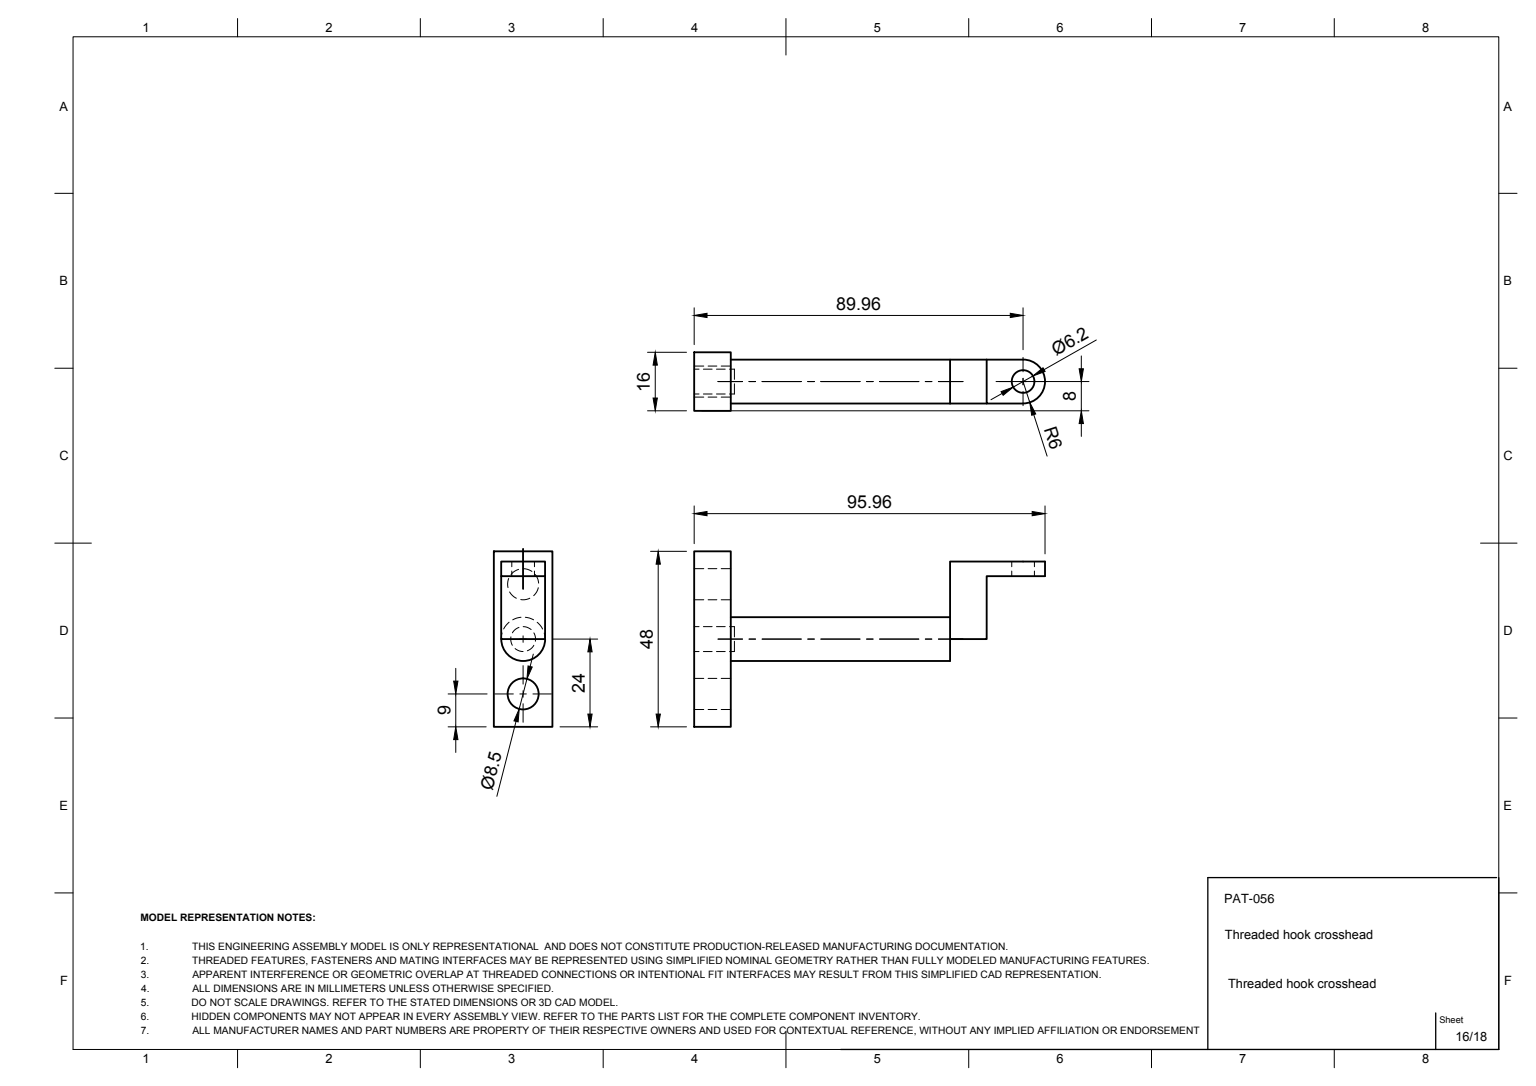
ISO-10303-21;
HEADER;
/* Generated by software containing ST-Developer
 * from STEP Tools, Inc. (www.steptools.com) 
 */

FILE_DESCRIPTION(
/* description */ ('Hook toggle clamp'),
/* implementation_level */ '2;1');

FILE_NAME(
/* name */ 'Threaded hook crosshead.step',
/* time_stamp */ '2026-10-27T21:56:56-07:00',
/* author */ (''),
/* organization */ (''),
/* preprocessor_version */ 'ST-DEVELOPER v20.2',
/* originating_system */ 'Autodesk Translation Framework v15.17.0.0',
/* authorisation */ '');

FILE_SCHEMA (('AUTOMOTIVE_DESIGN { 1 0 10303 214 3 1 1 }'));
ENDSEC;

DATA;
#10=MECHANICAL_DESIGN_GEOMETRIC_PRESENTATION_REPRESENTATION('',(#198),#5458);
#164=SHAPE_REPRESENTATION_RELATIONSHIP('SRR','None',#5548,#181);
#181=ADVANCED_BREP_SHAPE_REPRESENTATION('',(#214),#5450);
#198=STYLED_ITEM('',(#5731),#214);
#214=MANIFOLD_SOLID_BREP('Body1',#2980);
#259=FACE_BOUND('',#719,.T.);
#260=FACE_BOUND('',#720,.T.);
#261=FACE_BOUND('',#721,.T.);
#262=FACE_BOUND('',#727,.T.);
#263=FACE_BOUND('',#728,.T.);
#264=FACE_BOUND('',#729,.T.);
#265=FACE_BOUND('',#733,.T.);
#266=FACE_BOUND('',#740,.T.);
#356=PLANE('',#3372);
#357=PLANE('',#3379);
#358=PLANE('',#3381);
#359=PLANE('',#3382);
#360=PLANE('',#3383);
#361=PLANE('',#3384);
#362=PLANE('',#3385);
#363=PLANE('',#3392);
#364=PLANE('',#3393);
#365=PLANE('',#3394);
#366=PLANE('',#3395);
#367=PLANE('',#3396);
#368=PLANE('',#3397);
#369=PLANE('',#3399);
#370=PLANE('',#3400);
#504=FACE_OUTER_BOUND('',#714,.T.);
#505=FACE_OUTER_BOUND('',#715,.T.);
#506=FACE_OUTER_BOUND('',#716,.T.);
#507=FACE_OUTER_BOUND('',#717,.T.);
#508=FACE_OUTER_BOUND('',#718,.T.);
#509=FACE_OUTER_BOUND('',#722,.T.);
#510=FACE_OUTER_BOUND('',#723,.T.);
#511=FACE_OUTER_BOUND('',#724,.T.);
#512=FACE_OUTER_BOUND('',#725,.T.);
#513=FACE_OUTER_BOUND('',#726,.T.);
#514=FACE_OUTER_BOUND('',#730,.T.);
#515=FACE_OUTER_BOUND('',#731,.T.);
#516=FACE_OUTER_BOUND('',#732,.T.);
#517=FACE_OUTER_BOUND('',#734,.T.);
#518=FACE_OUTER_BOUND('',#735,.T.);
#519=FACE_OUTER_BOUND('',#736,.T.);
#520=FACE_OUTER_BOUND('',#737,.T.);
#521=FACE_OUTER_BOUND('',#738,.T.);
#522=FACE_OUTER_BOUND('',#739,.T.);
#523=FACE_OUTER_BOUND('',#741,.T.);
#524=FACE_OUTER_BOUND('',#742,.T.);
#714=EDGE_LOOP('',(#2497,#2498,#2499,#2500));
#715=EDGE_LOOP('',(#2501));
#716=EDGE_LOOP('',(#2502,#2503,#2504,#2505));
#717=EDGE_LOOP('',(#2506,#2507,#2508,#2509));
#718=EDGE_LOOP('',(#2510,#2511,#2512,#2513));
#719=EDGE_LOOP('',(#2514));
#720=EDGE_LOOP('',(#2515));
#721=EDGE_LOOP('',(#2516));
#722=EDGE_LOOP('',(#2517,#2518,#2519,#2520));
#723=EDGE_LOOP('',(#2521,#2522,#2523,#2524));
#724=EDGE_LOOP('',(#2525,#2526,#2527,#2528));
#725=EDGE_LOOP('',(#2529,#2530,#2531,#2532));
#726=EDGE_LOOP('',(#2533,#2534,#2535,#2536));
#727=EDGE_LOOP('',(#2537));
#728=EDGE_LOOP('',(#2538));
#729=EDGE_LOOP('',(#2539));
#730=EDGE_LOOP('',(#2540,#2541,#2542,#2543));
#731=EDGE_LOOP('',(#2544,#2545,#2546,#2547));
#732=EDGE_LOOP('',(#2548,#2549,#2550,#2551));
#733=EDGE_LOOP('',(#2552));
#734=EDGE_LOOP('',(#2553,#2554,#2555,#2556));
#735=EDGE_LOOP('',(#2557,#2558,#2559,#2560));
#736=EDGE_LOOP('',(#2561,#2562,#2563,#2564,#2565,#2566));
#737=EDGE_LOOP('',(#2567,#2568,#2569,#2570,#2571,#2572));
#738=EDGE_LOOP('',(#2573,#2574,#2575,#2576));
#739=EDGE_LOOP('',(#2577,#2578,#2579,#2580));
#740=EDGE_LOOP('',(#2581));
#741=EDGE_LOOP('',(#2582,#2583));
#742=EDGE_LOOP('',(#2584,#2585,#2586,#2587,#2588));
#971=LINE('',#4973,#1208);
#972=LINE('',#4980,#1209);
#973=LINE('',#4986,#1210);
#974=LINE('',#4991,#1211);
#975=LINE('',#4993,#1212);
#976=LINE('',#4995,#1213);
#977=LINE('',#4996,#1214);
#978=LINE('',#5001,#1215);
#979=LINE('',#5003,#1216);
#980=LINE('',#5004,#1217);
#981=LINE('',#5007,#1218);
#982=LINE('',#5008,#1219);
#983=LINE('',#5011,#1220);
#984=LINE('',#5012,#1221);
#985=LINE('',#5014,#1222);
#986=LINE('',#5020,#1223);
#987=LINE('',#5025,#1224);
#988=LINE('',#5029,#1225);
#989=LINE('',#5033,#1226);
#990=LINE('',#5035,#1227);
#991=LINE('',#5036,#1228);
#992=LINE('',#5039,#1229);
#993=LINE('',#5041,#1230);
#994=LINE('',#5042,#1231);
#995=LINE('',#5045,#1232);
#996=LINE('',#5047,#1233);
#997=LINE('',#5048,#1234);
#998=LINE('',#5051,#1235);
#999=LINE('',#5052,#1236);
#1000=LINE('',#5055,#1237);
#1001=LINE('',#5056,#1238);
#1002=LINE('',#5058,#1239);
#1003=LINE('',#5064,#1240);
#1208=VECTOR('',#4077,0.34);
#1209=VECTOR('',#4086,0.425);
#1210=VECTOR('',#4093,0.425);
#1211=VECTOR('',#4098,1.);
#1212=VECTOR('',#4099,1.);
#1213=VECTOR('',#4100,1.);
#1214=VECTOR('',#4101,1.);
#1215=VECTOR('',#4106,1.);
#1216=VECTOR('',#4107,1.);
#1217=VECTOR('',#4108,1.);
#1218=VECTOR('',#4111,1.);
#1219=VECTOR('',#4112,1.);
#1220=VECTOR('',#4115,1.);
#1221=VECTOR('',#4116,1.);
#1222=VECTOR('',#4119,1.);
#1223=VECTOR('',#4126,0.31);
#1224=VECTOR('',#4131,1.);
#1225=VECTOR('',#4134,1.);
#1226=VECTOR('',#4139,1.);
#1227=VECTOR('',#4140,1.);
#1228=VECTOR('',#4141,1.);
#1229=VECTOR('',#4144,1.);
#1230=VECTOR('',#4145,1.);
#1231=VECTOR('',#4146,1.);
#1232=VECTOR('',#4149,1.);
#1233=VECTOR('',#4150,1.);
#1234=VECTOR('',#4151,1.);
#1235=VECTOR('',#4154,1.);
#1236=VECTOR('',#4155,1.);
#1237=VECTOR('',#4158,1.);
#1238=VECTOR('',#4159,1.);
#1239=VECTOR('',#4162,1.);
#1240=VECTOR('',#4173,0.6);
#1335=CIRCLE('',#3370,0.34);
#1336=CIRCLE('',#3371,0.34);
#1337=CIRCLE('',#3374,0.425);
#1338=CIRCLE('',#3375,0.425);
#1339=CIRCLE('',#3377,0.425);
#1340=CIRCLE('',#3378,0.425);
#1341=CIRCLE('',#3380,0.6);
#1342=CIRCLE('',#3387,0.31);
#1343=CIRCLE('',#3388,0.31);
#1344=CIRCLE('',#3390,0.6);
#1345=CIRCLE('',#3391,0.6);
#1346=CIRCLE('',#3398,0.6);
#1347=CIRCLE('',#3401,0.6);
#1546=VERTEX_POINT('',#4970);
#1547=VERTEX_POINT('',#4972);
#1548=VERTEX_POINT('',#4977);
#1549=VERTEX_POINT('',#4979);
#1550=VERTEX_POINT('',#4983);
#1551=VERTEX_POINT('',#4985);
#1552=VERTEX_POINT('',#4989);
#1553=VERTEX_POINT('',#4990);
#1554=VERTEX_POINT('',#4992);
#1555=VERTEX_POINT('',#4994);
#1556=VERTEX_POINT('',#4997);
#1557=VERTEX_POINT('',#5000);
#1558=VERTEX_POINT('',#5002);
#1559=VERTEX_POINT('',#5006);
#1560=VERTEX_POINT('',#5010);
#1561=VERTEX_POINT('',#5017);
#1562=VERTEX_POINT('',#5019);
#1563=VERTEX_POINT('',#5023);
#1564=VERTEX_POINT('',#5024);
#1565=VERTEX_POINT('',#5026);
#1566=VERTEX_POINT('',#5028);
#1567=VERTEX_POINT('',#5032);
#1568=VERTEX_POINT('',#5034);
#1569=VERTEX_POINT('',#5038);
#1570=VERTEX_POINT('',#5040);
#1571=VERTEX_POINT('',#5044);
#1572=VERTEX_POINT('',#5046);
#1573=VERTEX_POINT('',#5050);
#1574=VERTEX_POINT('',#5054);
#1875=EDGE_CURVE('',#1546,#1546,#1335,.T.);
#1876=EDGE_CURVE('',#1546,#1547,#971,.T.);
#1877=EDGE_CURVE('',#1547,#1547,#1336,.T.);
#1878=EDGE_CURVE('',#1548,#1548,#1337,.T.);
#1879=EDGE_CURVE('',#1548,#1549,#972,.T.);
#1880=EDGE_CURVE('',#1549,#1549,#1338,.T.);
#1881=EDGE_CURVE('',#1550,#1550,#1339,.T.);
#1882=EDGE_CURVE('',#1550,#1551,#973,.T.);
#1883=EDGE_CURVE('',#1551,#1551,#1340,.T.);
#1884=EDGE_CURVE('',#1552,#1553,#974,.T.);
#1885=EDGE_CURVE('',#1554,#1552,#975,.T.);
#1886=EDGE_CURVE('',#1555,#1554,#976,.T.);
#1887=EDGE_CURVE('',#1553,#1555,#977,.T.);
#1888=EDGE_CURVE('',#1556,#1556,#1341,.T.);
#1889=EDGE_CURVE('',#1552,#1557,#978,.T.);
#1890=EDGE_CURVE('',#1558,#1557,#979,.T.);
#1891=EDGE_CURVE('',#1554,#1558,#980,.T.);
#1892=EDGE_CURVE('',#1559,#1558,#981,.T.);
#1893=EDGE_CURVE('',#1555,#1559,#982,.T.);
#1894=EDGE_CURVE('',#1560,#1559,#983,.T.);
#1895=EDGE_CURVE('',#1553,#1560,#984,.T.);
#1896=EDGE_CURVE('',#1557,#1560,#985,.T.);
#1897=EDGE_CURVE('',#1561,#1561,#1342,.T.);
#1898=EDGE_CURVE('',#1561,#1562,#986,.T.);
#1899=EDGE_CURVE('',#1562,#1562,#1343,.T.);
#1900=EDGE_CURVE('',#1563,#1564,#987,.T.);
#1901=EDGE_CURVE('',#1565,#1564,#1344,.T.);
#1902=EDGE_CURVE('',#1566,#1565,#988,.T.);
#1903=EDGE_CURVE('',#1566,#1563,#1345,.T.);
#1904=EDGE_CURVE('',#1566,#1567,#989,.T.);
#1905=EDGE_CURVE('',#1567,#1568,#990,.T.);
#1906=EDGE_CURVE('',#1568,#1563,#991,.T.);
#1907=EDGE_CURVE('',#1569,#1567,#992,.T.);
#1908=EDGE_CURVE('',#1570,#1569,#993,.T.);
#1909=EDGE_CURVE('',#1570,#1568,#994,.T.);
#1910=EDGE_CURVE('',#1571,#1570,#995,.T.);
#1911=EDGE_CURVE('',#1569,#1572,#996,.T.);
#1912=EDGE_CURVE('',#1571,#1572,#997,.T.);
#1913=EDGE_CURVE('',#1573,#1565,#998,.T.);
#1914=EDGE_CURVE('',#1572,#1573,#999,.T.);
#1915=EDGE_CURVE('',#1564,#1574,#1000,.T.);
#1916=EDGE_CURVE('',#1571,#1574,#1001,.T.);
#1917=EDGE_CURVE('',#1574,#1573,#1002,.T.);
#1918=EDGE_CURVE('',#1572,#1571,#1346,.T.);
#1919=EDGE_CURVE('',#1571,#1572,#1347,.T.);
#1920=EDGE_CURVE('',#1556,#1571,#1003,.T.);
#2497=ORIENTED_EDGE('',*,*,#1875,.F.);
#2498=ORIENTED_EDGE('',*,*,#1876,.T.);
#2499=ORIENTED_EDGE('',*,*,#1877,.F.);
#2500=ORIENTED_EDGE('',*,*,#1876,.F.);
#2501=ORIENTED_EDGE('',*,*,#1875,.T.);
#2502=ORIENTED_EDGE('',*,*,#1878,.F.);
#2503=ORIENTED_EDGE('',*,*,#1879,.T.);
#2504=ORIENTED_EDGE('',*,*,#1880,.F.);
#2505=ORIENTED_EDGE('',*,*,#1879,.F.);
#2506=ORIENTED_EDGE('',*,*,#1881,.F.);
#2507=ORIENTED_EDGE('',*,*,#1882,.T.);
#2508=ORIENTED_EDGE('',*,*,#1883,.F.);
#2509=ORIENTED_EDGE('',*,*,#1882,.F.);
#2510=ORIENTED_EDGE('',*,*,#1884,.F.);
#2511=ORIENTED_EDGE('',*,*,#1885,.F.);
#2512=ORIENTED_EDGE('',*,*,#1886,.F.);
#2513=ORIENTED_EDGE('',*,*,#1887,.F.);
#2514=ORIENTED_EDGE('',*,*,#1878,.T.);
#2515=ORIENTED_EDGE('',*,*,#1881,.T.);
#2516=ORIENTED_EDGE('',*,*,#1888,.T.);
#2517=ORIENTED_EDGE('',*,*,#1885,.T.);
#2518=ORIENTED_EDGE('',*,*,#1889,.T.);
#2519=ORIENTED_EDGE('',*,*,#1890,.F.);
#2520=ORIENTED_EDGE('',*,*,#1891,.F.);
#2521=ORIENTED_EDGE('',*,*,#1886,.T.);
#2522=ORIENTED_EDGE('',*,*,#1891,.T.);
#2523=ORIENTED_EDGE('',*,*,#1892,.F.);
#2524=ORIENTED_EDGE('',*,*,#1893,.F.);
#2525=ORIENTED_EDGE('',*,*,#1887,.T.);
#2526=ORIENTED_EDGE('',*,*,#1893,.T.);
#2527=ORIENTED_EDGE('',*,*,#1894,.F.);
#2528=ORIENTED_EDGE('',*,*,#1895,.F.);
#2529=ORIENTED_EDGE('',*,*,#1884,.T.);
#2530=ORIENTED_EDGE('',*,*,#1895,.T.);
#2531=ORIENTED_EDGE('',*,*,#1896,.F.);
#2532=ORIENTED_EDGE('',*,*,#1889,.F.);
#2533=ORIENTED_EDGE('',*,*,#1896,.T.);
#2534=ORIENTED_EDGE('',*,*,#1894,.T.);
#2535=ORIENTED_EDGE('',*,*,#1892,.T.);
#2536=ORIENTED_EDGE('',*,*,#1890,.T.);
#2537=ORIENTED_EDGE('',*,*,#1877,.T.);
#2538=ORIENTED_EDGE('',*,*,#1880,.T.);
#2539=ORIENTED_EDGE('',*,*,#1883,.T.);
#2540=ORIENTED_EDGE('',*,*,#1897,.F.);
#2541=ORIENTED_EDGE('',*,*,#1898,.T.);
#2542=ORIENTED_EDGE('',*,*,#1899,.F.);
#2543=ORIENTED_EDGE('',*,*,#1898,.F.);
#2544=ORIENTED_EDGE('',*,*,#1900,.T.);
#2545=ORIENTED_EDGE('',*,*,#1901,.F.);
#2546=ORIENTED_EDGE('',*,*,#1902,.F.);
#2547=ORIENTED_EDGE('',*,*,#1903,.T.);
#2548=ORIENTED_EDGE('',*,*,#1904,.T.);
#2549=ORIENTED_EDGE('',*,*,#1905,.T.);
#2550=ORIENTED_EDGE('',*,*,#1906,.T.);
#2551=ORIENTED_EDGE('',*,*,#1903,.F.);
#2552=ORIENTED_EDGE('',*,*,#1897,.T.);
#2553=ORIENTED_EDGE('',*,*,#1905,.F.);
#2554=ORIENTED_EDGE('',*,*,#1907,.F.);
#2555=ORIENTED_EDGE('',*,*,#1908,.F.);
#2556=ORIENTED_EDGE('',*,*,#1909,.T.);
#2557=ORIENTED_EDGE('',*,*,#1910,.T.);
#2558=ORIENTED_EDGE('',*,*,#1908,.T.);
#2559=ORIENTED_EDGE('',*,*,#1911,.T.);
#2560=ORIENTED_EDGE('',*,*,#1912,.F.);
#2561=ORIENTED_EDGE('',*,*,#1904,.F.);
#2562=ORIENTED_EDGE('',*,*,#1902,.T.);
#2563=ORIENTED_EDGE('',*,*,#1913,.F.);
#2564=ORIENTED_EDGE('',*,*,#1914,.F.);
#2565=ORIENTED_EDGE('',*,*,#1911,.F.);
#2566=ORIENTED_EDGE('',*,*,#1907,.T.);
#2567=ORIENTED_EDGE('',*,*,#1915,.F.);
#2568=ORIENTED_EDGE('',*,*,#1900,.F.);
#2569=ORIENTED_EDGE('',*,*,#1906,.F.);
#2570=ORIENTED_EDGE('',*,*,#1909,.F.);
#2571=ORIENTED_EDGE('',*,*,#1910,.F.);
#2572=ORIENTED_EDGE('',*,*,#1916,.T.);
#2573=ORIENTED_EDGE('',*,*,#1914,.T.);
#2574=ORIENTED_EDGE('',*,*,#1917,.F.);
#2575=ORIENTED_EDGE('',*,*,#1916,.F.);
#2576=ORIENTED_EDGE('',*,*,#1918,.F.);
#2577=ORIENTED_EDGE('',*,*,#1915,.T.);
#2578=ORIENTED_EDGE('',*,*,#1917,.T.);
#2579=ORIENTED_EDGE('',*,*,#1913,.T.);
#2580=ORIENTED_EDGE('',*,*,#1901,.T.);
#2581=ORIENTED_EDGE('',*,*,#1899,.T.);
#2582=ORIENTED_EDGE('',*,*,#1912,.T.);
#2583=ORIENTED_EDGE('',*,*,#1919,.F.);
#2584=ORIENTED_EDGE('',*,*,#1888,.F.);
#2585=ORIENTED_EDGE('',*,*,#1920,.T.);
#2586=ORIENTED_EDGE('',*,*,#1919,.T.);
#2587=ORIENTED_EDGE('',*,*,#1918,.T.);
#2588=ORIENTED_EDGE('',*,*,#1920,.F.);
#2778=CYLINDRICAL_SURFACE('',#3369,0.34);
#2779=CYLINDRICAL_SURFACE('',#3373,0.425);
#2780=CYLINDRICAL_SURFACE('',#3376,0.425);
#2781=CYLINDRICAL_SURFACE('',#3386,0.31);
#2782=CYLINDRICAL_SURFACE('',#3389,0.6);
#2783=CYLINDRICAL_SURFACE('',#3402,0.6);
#2908=ADVANCED_FACE('',(#504),#2778,.F.);
#2909=ADVANCED_FACE('',(#505),#356,.T.);
#2910=ADVANCED_FACE('',(#506),#2779,.F.);
#2911=ADVANCED_FACE('',(#507),#2780,.F.);
#2912=ADVANCED_FACE('',(#508,#259,#260,#261),#357,.F.);
#2913=ADVANCED_FACE('',(#509),#358,.T.);
#2914=ADVANCED_FACE('',(#510),#359,.T.);
#2915=ADVANCED_FACE('',(#511),#360,.T.);
#2916=ADVANCED_FACE('',(#512),#361,.T.);
#2917=ADVANCED_FACE('',(#513,#262,#263,#264),#362,.T.);
#2918=ADVANCED_FACE('',(#514),#2781,.F.);
#2919=ADVANCED_FACE('',(#515),#2782,.T.);
#2920=ADVANCED_FACE('',(#516,#265),#363,.F.);
#2921=ADVANCED_FACE('',(#517),#364,.T.);
#2922=ADVANCED_FACE('',(#518),#365,.F.);
#2923=ADVANCED_FACE('',(#519),#366,.T.);
#2924=ADVANCED_FACE('',(#520),#367,.T.);
#2925=ADVANCED_FACE('',(#521),#368,.T.);
#2926=ADVANCED_FACE('',(#522,#266),#369,.T.);
#2927=ADVANCED_FACE('',(#523),#370,.F.);
#2928=ADVANCED_FACE('',(#524),#2783,.T.);
#2980=CLOSED_SHELL('',(#2908,#2909,#2910,#2911,#2912,#2913,#2914,#2915,
#2916,#2917,#2918,#2919,#2920,#2921,#2922,#2923,#2924,#2925,#2926,#2927,
#2928));
#3368=AXIS2_PLACEMENT_3D('',#4968,#4071,#4072);
#3369=AXIS2_PLACEMENT_3D('',#4969,#4073,#4074);
#3370=AXIS2_PLACEMENT_3D('',#4971,#4075,#4076);
#3371=AXIS2_PLACEMENT_3D('',#4974,#4078,#4079);
#3372=AXIS2_PLACEMENT_3D('',#4975,#4080,#4081);
#3373=AXIS2_PLACEMENT_3D('',#4976,#4082,#4083);
#3374=AXIS2_PLACEMENT_3D('',#4978,#4084,#4085);
#3375=AXIS2_PLACEMENT_3D('',#4981,#4087,#4088);
#3376=AXIS2_PLACEMENT_3D('',#4982,#4089,#4090);
#3377=AXIS2_PLACEMENT_3D('',#4984,#4091,#4092);
#3378=AXIS2_PLACEMENT_3D('',#4987,#4094,#4095);
#3379=AXIS2_PLACEMENT_3D('',#4988,#4096,#4097);
#3380=AXIS2_PLACEMENT_3D('',#4998,#4102,#4103);
#3381=AXIS2_PLACEMENT_3D('',#4999,#4104,#4105);
#3382=AXIS2_PLACEMENT_3D('',#5005,#4109,#4110);
#3383=AXIS2_PLACEMENT_3D('',#5009,#4113,#4114);
#3384=AXIS2_PLACEMENT_3D('',#5013,#4117,#4118);
#3385=AXIS2_PLACEMENT_3D('',#5015,#4120,#4121);
#3386=AXIS2_PLACEMENT_3D('',#5016,#4122,#4123);
#3387=AXIS2_PLACEMENT_3D('',#5018,#4124,#4125);
#3388=AXIS2_PLACEMENT_3D('',#5021,#4127,#4128);
#3389=AXIS2_PLACEMENT_3D('',#5022,#4129,#4130);
#3390=AXIS2_PLACEMENT_3D('',#5027,#4132,#4133);
#3391=AXIS2_PLACEMENT_3D('',#5030,#4135,#4136);
#3392=AXIS2_PLACEMENT_3D('',#5031,#4137,#4138);
#3393=AXIS2_PLACEMENT_3D('',#5037,#4142,#4143);
#3394=AXIS2_PLACEMENT_3D('',#5043,#4147,#4148);
#3395=AXIS2_PLACEMENT_3D('',#5049,#4152,#4153);
#3396=AXIS2_PLACEMENT_3D('',#5053,#4156,#4157);
#3397=AXIS2_PLACEMENT_3D('',#5057,#4160,#4161);
#3398=AXIS2_PLACEMENT_3D('',#5059,#4163,#4164);
#3399=AXIS2_PLACEMENT_3D('',#5060,#4165,#4166);
#3400=AXIS2_PLACEMENT_3D('',#5061,#4167,#4168);
#3401=AXIS2_PLACEMENT_3D('',#5062,#4169,#4170);
#3402=AXIS2_PLACEMENT_3D('',#5063,#4171,#4172);
#4071=DIRECTION('axis',(0.,0.,1.));
#4072=DIRECTION('refdir',(1.,0.,0.));
#4073=DIRECTION('center_axis',(1.,0.,0.));
#4074=DIRECTION('ref_axis',(0.,0.,-1.));
#4075=DIRECTION('center_axis',(1.,0.,0.));
#4076=DIRECTION('ref_axis',(0.,0.,-1.));
#4077=DIRECTION('',(1.,0.,0.));
#4078=DIRECTION('center_axis',(-1.,0.,0.));
#4079=DIRECTION('ref_axis',(0.,0.,-1.));
#4080=DIRECTION('center_axis',(1.,0.,0.));
#4081=DIRECTION('ref_axis',(0.,0.,-1.));
#4082=DIRECTION('center_axis',(1.,0.,0.));
#4083=DIRECTION('ref_axis',(0.,0.,-1.));
#4084=DIRECTION('center_axis',(1.,0.,0.));
#4085=DIRECTION('ref_axis',(0.,0.,-1.));
#4086=DIRECTION('',(1.,0.,0.));
#4087=DIRECTION('center_axis',(-1.,0.,0.));
#4088=DIRECTION('ref_axis',(0.,0.,-1.));
#4089=DIRECTION('center_axis',(1.,0.,0.));
#4090=DIRECTION('ref_axis',(0.,0.,-1.));
#4091=DIRECTION('center_axis',(1.,0.,0.));
#4092=DIRECTION('ref_axis',(0.,0.,-1.));
#4093=DIRECTION('',(1.,0.,0.));
#4094=DIRECTION('center_axis',(-1.,0.,0.));
#4095=DIRECTION('ref_axis',(0.,0.,-1.));
#4096=DIRECTION('center_axis',(1.,0.,0.));
#4097=DIRECTION('ref_axis',(0.,0.,-1.));
#4098=DIRECTION('',(0.,0.,-1.));
#4099=DIRECTION('',(0.,-1.,0.));
#4100=DIRECTION('',(0.,0.,1.));
#4101=DIRECTION('',(0.,1.,0.));
#4102=DIRECTION('center_axis',(1.,0.,0.));
#4103=DIRECTION('ref_axis',(0.,0.,-1.));
#4104=DIRECTION('center_axis',(0.,0.,1.));
#4105=DIRECTION('ref_axis',(0.,-1.,0.));
#4106=DIRECTION('',(1.,0.,0.));
#4107=DIRECTION('',(0.,-1.,0.));
#4108=DIRECTION('',(1.,0.,0.));
#4109=DIRECTION('center_axis',(0.,1.,0.));
#4110=DIRECTION('ref_axis',(0.,0.,1.));
#4111=DIRECTION('',(0.,0.,1.));
#4112=DIRECTION('',(1.,0.,0.));
#4113=DIRECTION('center_axis',(0.,0.,-1.));
#4114=DIRECTION('ref_axis',(0.,1.,0.));
#4115=DIRECTION('',(0.,1.,0.));
#4116=DIRECTION('',(1.,0.,0.));
#4117=DIRECTION('center_axis',(0.,-1.,0.));
#4118=DIRECTION('ref_axis',(0.,0.,-1.));
#4119=DIRECTION('',(0.,0.,-1.));
#4120=DIRECTION('center_axis',(1.,0.,0.));
#4121=DIRECTION('ref_axis',(0.,0.,-1.));
#4122=DIRECTION('center_axis',(0.,1.,0.));
#4123=DIRECTION('ref_axis',(1.,0.,0.));
#4124=DIRECTION('center_axis',(0.,1.,0.));
#4125=DIRECTION('ref_axis',(1.,0.,0.));
#4126=DIRECTION('',(0.,1.,0.));
#4127=DIRECTION('center_axis',(0.,-1.,0.));
#4128=DIRECTION('ref_axis',(1.,0.,0.));
#4129=DIRECTION('center_axis',(0.,1.,0.));
#4130=DIRECTION('ref_axis',(-1.,0.,1.22464679914735E-16));
#4131=DIRECTION('',(0.,1.,0.));
#4132=DIRECTION('center_axis',(0.,1.,0.));
#4133=DIRECTION('ref_axis',(1.,0.,0.));
#4134=DIRECTION('',(0.,1.,0.));
#4135=DIRECTION('center_axis',(0.,1.,0.));
#4136=DIRECTION('ref_axis',(1.,0.,0.));
#4137=DIRECTION('center_axis',(0.,1.,0.));
#4138=DIRECTION('ref_axis',(1.,0.,0.));
#4139=DIRECTION('',(1.,0.,0.));
#4140=DIRECTION('',(0.,0.,1.));
#4141=DIRECTION('',(-1.,0.,0.));
#4142=DIRECTION('center_axis',(-1.,0.,0.));
#4143=DIRECTION('ref_axis',(0.,0.,1.));
#4144=DIRECTION('',(0.,1.,0.));
#4145=DIRECTION('',(0.,0.,-1.));
#4146=DIRECTION('',(0.,1.,0.));
#4147=DIRECTION('center_axis',(0.,1.,0.));
#4148=DIRECTION('ref_axis',(1.,0.,0.));
#4149=DIRECTION('',(-1.,0.,0.));
#4150=DIRECTION('',(1.,0.,0.));
#4151=DIRECTION('',(0.,0.,-1.));
#4152=DIRECTION('center_axis',(0.,0.,-1.));
#4153=DIRECTION('ref_axis',(-1.,0.,0.));
#4154=DIRECTION('',(-1.,0.,0.));
#4155=DIRECTION('',(0.,1.,0.));
#4156=DIRECTION('center_axis',(0.,0.,1.));
#4157=DIRECTION('ref_axis',(1.,0.,0.));
#4158=DIRECTION('',(1.,0.,0.));
#4159=DIRECTION('',(0.,1.,0.));
#4160=DIRECTION('center_axis',(1.,0.,0.));
#4161=DIRECTION('ref_axis',(0.,0.,-1.));
#4162=DIRECTION('',(0.,0.,-1.));
#4163=DIRECTION('center_axis',(1.,0.,0.));
#4164=DIRECTION('ref_axis',(0.,0.,-1.));
#4165=DIRECTION('center_axis',(0.,1.,0.));
#4166=DIRECTION('ref_axis',(0.,0.,1.));
#4167=DIRECTION('center_axis',(1.,0.,0.));
#4168=DIRECTION('ref_axis',(0.,0.,-1.));
#4169=DIRECTION('center_axis',(1.,0.,0.));
#4170=DIRECTION('ref_axis',(0.,0.,-1.));
#4171=DIRECTION('center_axis',(1.,0.,0.));
#4172=DIRECTION('ref_axis',(0.,0.,-1.));
#4173=DIRECTION('',(-1.,0.,0.));
#4968=CARTESIAN_POINT('',(0.,0.,0.));
#4969=CARTESIAN_POINT('Origin',(9.9,0.,2.5));
#4970=CARTESIAN_POINT('',(9.9,-4.163799117101E-17,2.84));
#4971=CARTESIAN_POINT('Origin',(9.9,0.,2.5));
#4972=CARTESIAN_POINT('',(11.,4.163799117101E-17,2.84));
#4973=CARTESIAN_POINT('',(9.9,-4.163799117101E-17,2.84));
#4974=CARTESIAN_POINT('Origin',(11.,0.,2.5));
#4975=CARTESIAN_POINT('Origin',(9.9,0.,2.5));
#4976=CARTESIAN_POINT('Origin',(9.9,-1.5,2.5));
#4977=CARTESIAN_POINT('',(10.,-1.5,2.925));
#4978=CARTESIAN_POINT('Origin',(10.,-1.5,2.5));
#4979=CARTESIAN_POINT('',(11.,-1.5,2.925));
#4980=CARTESIAN_POINT('',(9.9,-1.5,2.925));
#4981=CARTESIAN_POINT('Origin',(11.,-1.5,2.5));
#4982=CARTESIAN_POINT('Origin',(9.9,1.5,2.5));
#4983=CARTESIAN_POINT('',(10.,1.5,2.925));
#4984=CARTESIAN_POINT('Origin',(10.,1.5,2.5));
#4985=CARTESIAN_POINT('',(11.,1.5,2.925));
#4986=CARTESIAN_POINT('',(9.9,1.5,2.925));
#4987=CARTESIAN_POINT('Origin',(11.,1.5,2.5));
#4988=CARTESIAN_POINT('Origin',(10.,0.,2.5));
#4989=CARTESIAN_POINT('',(10.,-2.4,3.3));
#4990=CARTESIAN_POINT('',(10.,-2.4,1.7));
#4991=CARTESIAN_POINT('',(10.,-2.4,3.3));
#4992=CARTESIAN_POINT('',(10.,2.4,3.3));
#4993=CARTESIAN_POINT('',(10.,2.4,3.3));
#4994=CARTESIAN_POINT('',(10.,2.4,1.7));
#4995=CARTESIAN_POINT('',(10.,2.4,1.7));
#4996=CARTESIAN_POINT('',(10.,-2.4,1.7));
#4997=CARTESIAN_POINT('',(10.,-7.34788079488412E-17,3.1));
#4998=CARTESIAN_POINT('Origin',(10.,0.,2.5));
#4999=CARTESIAN_POINT('Origin',(10.,2.4,3.3));
#5000=CARTESIAN_POINT('',(11.,-2.4,3.3));
#5001=CARTESIAN_POINT('',(10.,-2.4,3.3));
#5002=CARTESIAN_POINT('',(11.,2.4,3.3));
#5003=CARTESIAN_POINT('',(11.,2.4,3.3));
#5004=CARTESIAN_POINT('',(10.,2.4,3.3));
#5005=CARTESIAN_POINT('Origin',(10.,2.4,1.7));
#5006=CARTESIAN_POINT('',(11.,2.4,1.7));
#5007=CARTESIAN_POINT('',(11.,2.4,1.7));
#5008=CARTESIAN_POINT('',(10.,2.4,1.7));
#5009=CARTESIAN_POINT('Origin',(10.,-2.4,1.7));
#5010=CARTESIAN_POINT('',(11.,-2.4,1.7));
#5011=CARTESIAN_POINT('',(11.,-2.4,1.7));
#5012=CARTESIAN_POINT('',(10.,-2.4,1.7));
#5013=CARTESIAN_POINT('Origin',(10.,-2.4,3.3));
#5014=CARTESIAN_POINT('',(11.,-2.4,3.3));
#5015=CARTESIAN_POINT('Origin',(11.,0.,2.5));
#5016=CARTESIAN_POINT('Origin',(2.00423507354465,1.6,2.5));
#5017=CARTESIAN_POINT('',(1.69423507354465,1.72,2.5));
#5018=CARTESIAN_POINT('Origin',(2.00423507354465,1.72,2.5));
#5019=CARTESIAN_POINT('',(1.69423507354465,2.12,2.5));
#5020=CARTESIAN_POINT('',(1.69423507354465,1.6,2.5));
#5021=CARTESIAN_POINT('Origin',(2.00423507354465,2.12,2.5));
#5022=CARTESIAN_POINT('Origin',(2.00423507354465,1.72,2.5));
#5023=CARTESIAN_POINT('',(2.00423507354465,1.72,3.1));
#5024=CARTESIAN_POINT('',(2.00423507354465,2.12,3.1));
#5025=CARTESIAN_POINT('',(2.00423507354465,1.72,3.1));
#5026=CARTESIAN_POINT('',(2.00423507354465,2.12,1.9));
#5027=CARTESIAN_POINT('Origin',(2.00423507354465,2.12,2.5));
#5028=CARTESIAN_POINT('',(2.00423507354465,1.72,1.9));
#5029=CARTESIAN_POINT('',(2.00423507354465,1.72,1.9));
#5030=CARTESIAN_POINT('Origin',(2.00423507354465,1.72,2.5));
#5031=CARTESIAN_POINT('Origin',(3.00211753677232,1.72,2.5));
#5032=CARTESIAN_POINT('',(3.,1.72,1.9));
#5033=CARTESIAN_POINT('',(2.00423507354465,1.72,1.9));
#5034=CARTESIAN_POINT('',(3.,1.72,3.1));
#5035=CARTESIAN_POINT('',(3.,1.72,2.2));
#5036=CARTESIAN_POINT('',(4.,1.72,3.1));
#5037=CARTESIAN_POINT('Origin',(3.,0.,1.9));
#5038=CARTESIAN_POINT('',(3.,0.,1.9));
#5039=CARTESIAN_POINT('',(3.,0.,1.9));
#5040=CARTESIAN_POINT('',(3.,0.,3.1));
#5041=CARTESIAN_POINT('',(3.,0.,3.1));
#5042=CARTESIAN_POINT('',(3.,0.,3.1));
#5043=CARTESIAN_POINT('Origin',(3.5,0.,2.5));
#5044=CARTESIAN_POINT('',(4.,-7.34788079488412E-17,3.1));
#5045=CARTESIAN_POINT('',(4.,0.,3.1));
#5046=CARTESIAN_POINT('',(4.,0.,1.9));
#5047=CARTESIAN_POINT('',(3.,0.,1.9));
#5048=CARTESIAN_POINT('',(4.,0.,2.5));
#5049=CARTESIAN_POINT('Origin',(4.,1.72,1.9));
#5050=CARTESIAN_POINT('',(4.,2.12,1.9));
#5051=CARTESIAN_POINT('',(2.00423507354465,2.12,1.9));
#5052=CARTESIAN_POINT('',(4.,1.72,1.9));
#5053=CARTESIAN_POINT('Origin',(2.00423507354465,1.72,3.1));
#5054=CARTESIAN_POINT('',(4.,2.12,3.1));
#5055=CARTESIAN_POINT('',(4.,2.12,3.1));
#5056=CARTESIAN_POINT('',(4.,1.72,3.1));
#5057=CARTESIAN_POINT('Origin',(4.,1.72,3.1));
#5058=CARTESIAN_POINT('',(4.,2.12,1.9));
#5059=CARTESIAN_POINT('Origin',(4.,0.,2.5));
#5060=CARTESIAN_POINT('Origin',(3.00211753677232,2.12,2.5));
#5061=CARTESIAN_POINT('Origin',(4.,0.,2.5));
#5062=CARTESIAN_POINT('Origin',(4.,0.,2.5));
#5063=CARTESIAN_POINT('Origin',(4.,0.,2.5));
#5064=CARTESIAN_POINT('',(4.,-7.34788079488412E-17,3.1));
#5427=UNCERTAINTY_MEASURE_WITH_UNIT(LENGTH_MEASURE(0.001),#5459,
'DISTANCE_ACCURACY_VALUE',
'Maximum model space distance between geometric entities at asserted c
onnectivities');
#5435=UNCERTAINTY_MEASURE_WITH_UNIT(LENGTH_MEASURE(0.001),#5459,
'DISTANCE_ACCURACY_VALUE',
'Maximum model space distance between geometric entities at asserted c
onnectivities');
#5450=(
GEOMETRIC_REPRESENTATION_CONTEXT(3)
GLOBAL_UNCERTAINTY_ASSIGNED_CONTEXT((#5427))
GLOBAL_UNIT_ASSIGNED_CONTEXT((#5459,#5461,#5462))
REPRESENTATION_CONTEXT('','3D')
);
#5458=(
GEOMETRIC_REPRESENTATION_CONTEXT(3)
GLOBAL_UNCERTAINTY_ASSIGNED_CONTEXT((#5435))
GLOBAL_UNIT_ASSIGNED_CONTEXT((#5459,#5461,#5462))
REPRESENTATION_CONTEXT('','3D')
);
#5459=(
LENGTH_UNIT()
NAMED_UNIT(*)
SI_UNIT(.CENTI.,.METRE.)
);
#5461=(
NAMED_UNIT(*)
PLANE_ANGLE_UNIT()
SI_UNIT($,.RADIAN.)
);
#5462=(
NAMED_UNIT(*)
SI_UNIT($,.STERADIAN.)
SOLID_ANGLE_UNIT()
);
#5477=SHAPE_DEFINITION_REPRESENTATION(#5500,#5548);
#5500=PRODUCT_DEFINITION_SHAPE('',$,#5571);
#5548=SHAPE_REPRESENTATION('',(#3368),#5450);
#5556=PRODUCT_DEFINITION_CONTEXT('part definition',#5624,'design');
#5571=PRODUCT_DEFINITION('Threaded hook crosshead',
'Threaded hook crosshead',#5593,#5556);
#5593=PRODUCT_DEFINITION_FORMATION('',$,#5640);
#5624=APPLICATION_CONTEXT(
'Core Data for Automotive Mechanical Design Process');
#5625=PRODUCT_CONTEXT('part definition',#5624,'mechanical');
#5640=PRODUCT('Threaded hook crosshead','Threaded hook crosshead',
'Threaded hook crosshead',(#5625));
#5725=COLOUR_RGB('Off White',0.89,0.88,0.83);
#5726=FILL_AREA_STYLE_COLOUR('',#5725);
#5727=FILL_AREA_STYLE('',(#5726));
#5728=SURFACE_STYLE_FILL_AREA(#5727);
#5729=SURFACE_SIDE_STYLE('',(#5728));
#5730=SURFACE_STYLE_USAGE(.BOTH.,#5729);
#5731=PRESENTATION_STYLE_ASSIGNMENT((#5730));
ENDSEC;
END-ISO-10303-21;
